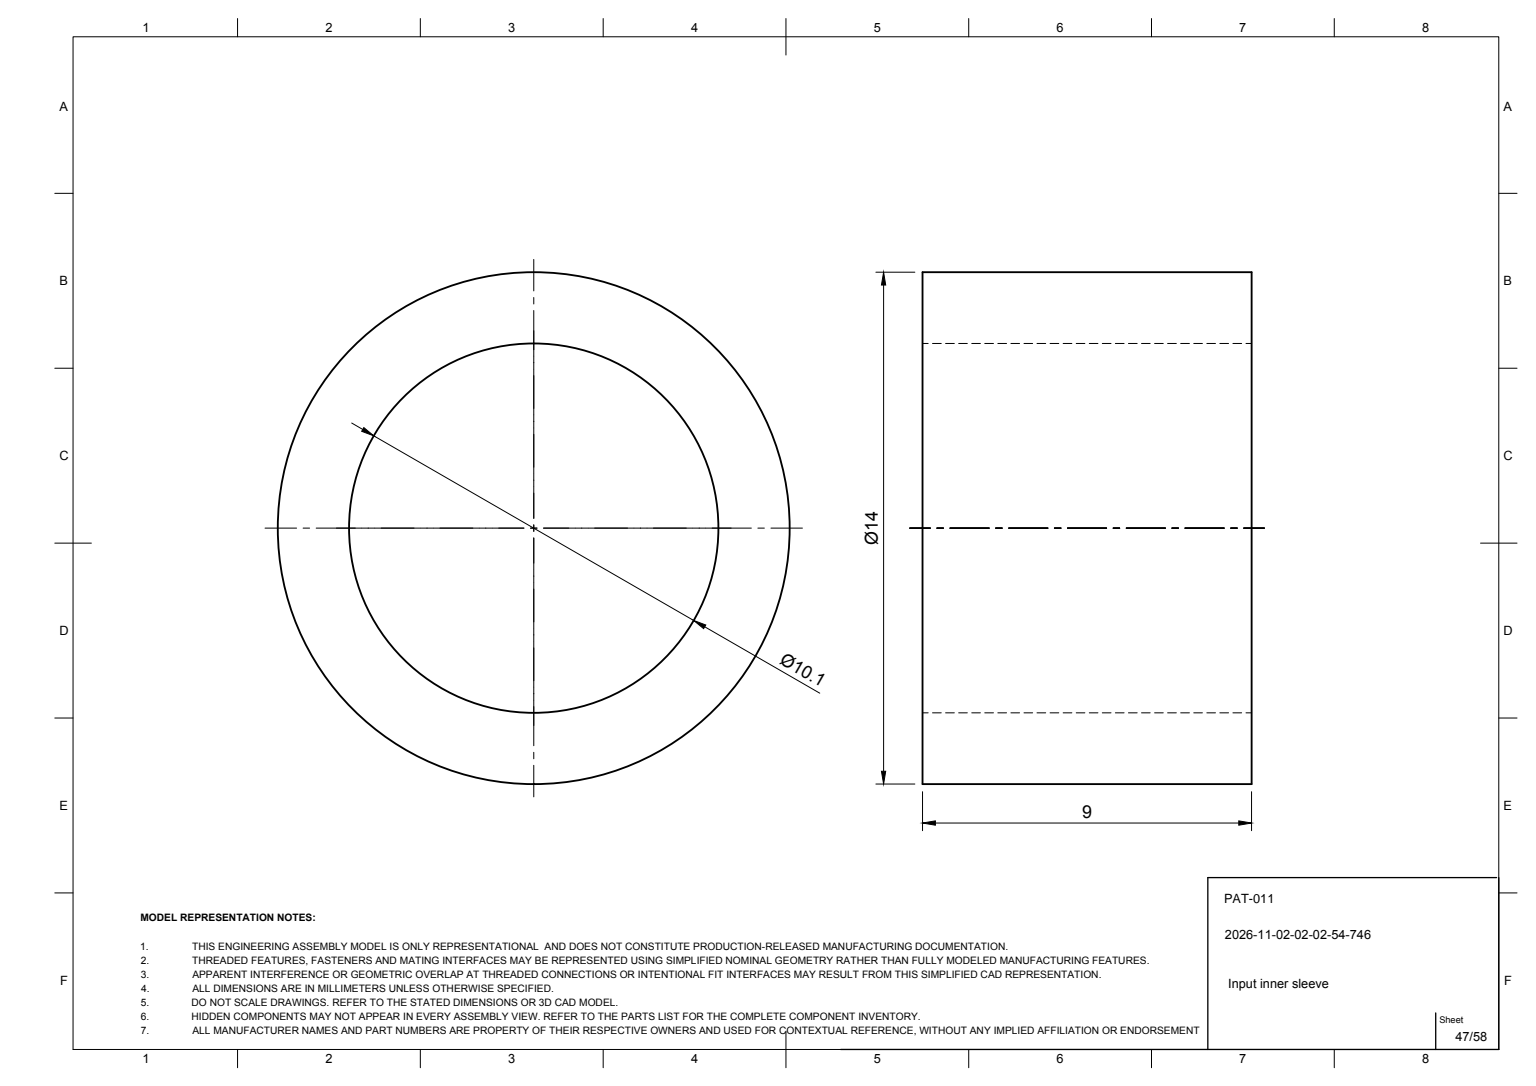
ISO-10303-21;
HEADER;
/* Generated by software containing ST-Developer
 * from STEP Tools, Inc. (www.steptools.com) 
 */

FILE_DESCRIPTION(
/* description */ ('Belt tension measurement rig'),
/* implementation_level */ '2;1');

FILE_NAME(
/* name */ 'Input inner sleeve.step',
/* time_stamp */ '2026-10-28T03:24:44-07:00',
/* author */ (''),
/* organization */ (''),
/* preprocessor_version */ 'ST-DEVELOPER v20.2',
/* originating_system */ 'Autodesk Translation Framework v15.17.0.0',
/* authorisation */ '');

FILE_SCHEMA (('AUTOMOTIVE_DESIGN { 1 0 10303 214 3 1 1 }'));
ENDSEC;

DATA;
#10=MECHANICAL_DESIGN_GEOMETRIC_PRESENTATION_REPRESENTATION('',(#746),#23587);
#621=SHAPE_REPRESENTATION_RELATIONSHIP('SRR','None',#23871,#676);
#676=ADVANCED_BREP_SHAPE_REPRESENTATION('',(#814),#23569);
#746=STYLED_ITEM('',(#24197),#814);
#814=MANIFOLD_SOLID_BREP('Body1',#12253);
#991=FACE_BOUND('',#2685,.T.);
#992=FACE_BOUND('',#2687,.T.);
#1286=PLANE('',#13848);
#1287=PLANE('',#13849);
#1816=FACE_OUTER_BOUND('',#2682,.T.);
#1817=FACE_OUTER_BOUND('',#2683,.T.);
#1818=FACE_OUTER_BOUND('',#2684,.T.);
#1819=FACE_OUTER_BOUND('',#2686,.T.);
#2682=EDGE_LOOP('',(#9968,#9969,#9970,#9971));
#2683=EDGE_LOOP('',(#9972,#9973,#9974,#9975));
#2684=EDGE_LOOP('',(#9976));
#2685=EDGE_LOOP('',(#9977));
#2686=EDGE_LOOP('',(#9978));
#2687=EDGE_LOOP('',(#9979));
#3501=LINE('',#21506,#4252);
#3502=LINE('',#21512,#4253);
#4252=VECTOR('',#16986,0.505);
#4253=VECTOR('',#16993,0.7);
#4912=CIRCLE('',#13843,0.505);
#4913=CIRCLE('',#13844,0.505);
#4914=CIRCLE('',#13846,0.7);
#4915=CIRCLE('',#13847,0.7);
#5927=VERTEX_POINT('',#21503);
#5928=VERTEX_POINT('',#21505);
#5929=VERTEX_POINT('',#21509);
#5930=VERTEX_POINT('',#21511);
#7343=EDGE_CURVE('',#5927,#5927,#4912,.T.);
#7344=EDGE_CURVE('',#5927,#5928,#3501,.T.);
#7345=EDGE_CURVE('',#5928,#5928,#4913,.T.);
#7346=EDGE_CURVE('',#5929,#5929,#4914,.T.);
#7347=EDGE_CURVE('',#5929,#5930,#3502,.T.);
#7348=EDGE_CURVE('',#5930,#5930,#4915,.T.);
#9968=ORIENTED_EDGE('',*,*,#7343,.F.);
#9969=ORIENTED_EDGE('',*,*,#7344,.T.);
#9970=ORIENTED_EDGE('',*,*,#7345,.T.);
#9971=ORIENTED_EDGE('',*,*,#7344,.F.);
#9972=ORIENTED_EDGE('',*,*,#7346,.F.);
#9973=ORIENTED_EDGE('',*,*,#7347,.T.);
#9974=ORIENTED_EDGE('',*,*,#7348,.T.);
#9975=ORIENTED_EDGE('',*,*,#7347,.F.);
#9976=ORIENTED_EDGE('',*,*,#7346,.T.);
#9977=ORIENTED_EDGE('',*,*,#7343,.T.);
#9978=ORIENTED_EDGE('',*,*,#7348,.F.);
#9979=ORIENTED_EDGE('',*,*,#7345,.F.);
#11325=CYLINDRICAL_SURFACE('',#13842,0.505);
#11326=CYLINDRICAL_SURFACE('',#13845,0.7);
#11957=ADVANCED_FACE('',(#1816),#11325,.F.);
#11958=ADVANCED_FACE('',(#1817),#11326,.T.);
#11959=ADVANCED_FACE('',(#1818,#991),#1286,.T.);
#11960=ADVANCED_FACE('',(#1819,#992),#1287,.F.);
#12253=CLOSED_SHELL('',(#11957,#11958,#11959,#11960));
#13841=AXIS2_PLACEMENT_3D('',#21501,#16980,#16981);
#13842=AXIS2_PLACEMENT_3D('',#21502,#16982,#16983);
#13843=AXIS2_PLACEMENT_3D('',#21504,#16984,#16985);
#13844=AXIS2_PLACEMENT_3D('',#21507,#16987,#16988);
#13845=AXIS2_PLACEMENT_3D('',#21508,#16989,#16990);
#13846=AXIS2_PLACEMENT_3D('',#21510,#16991,#16992);
#13847=AXIS2_PLACEMENT_3D('',#21513,#16994,#16995);
#13848=AXIS2_PLACEMENT_3D('',#21514,#16996,#16997);
#13849=AXIS2_PLACEMENT_3D('',#21515,#16998,#16999);
#16980=DIRECTION('axis',(0.,0.,1.));
#16981=DIRECTION('refdir',(1.,0.,0.));
#16982=DIRECTION('center_axis',(0.,1.,0.));
#16983=DIRECTION('ref_axis',(1.,0.,0.));
#16984=DIRECTION('center_axis',(0.,-1.,0.));
#16985=DIRECTION('ref_axis',(1.,0.,0.));
#16986=DIRECTION('',(0.,-1.,0.));
#16987=DIRECTION('center_axis',(0.,-1.,0.));
#16988=DIRECTION('ref_axis',(1.,0.,0.));
#16989=DIRECTION('center_axis',(0.,1.,0.));
#16990=DIRECTION('ref_axis',(1.,0.,0.));
#16991=DIRECTION('center_axis',(0.,1.,0.));
#16992=DIRECTION('ref_axis',(1.,0.,0.));
#16993=DIRECTION('',(0.,-1.,0.));
#16994=DIRECTION('center_axis',(0.,1.,0.));
#16995=DIRECTION('ref_axis',(1.,0.,0.));
#16996=DIRECTION('center_axis',(0.,1.,0.));
#16997=DIRECTION('ref_axis',(1.,0.,0.));
#16998=DIRECTION('center_axis',(0.,1.,0.));
#16999=DIRECTION('ref_axis',(1.,0.,0.));
#21501=CARTESIAN_POINT('',(0.,0.,0.));
#21502=CARTESIAN_POINT('Origin',(0.,-0.45,7.));
#21503=CARTESIAN_POINT('',(-0.505,0.45,7.));
#21504=CARTESIAN_POINT('Origin',(0.,0.45,7.));
#21505=CARTESIAN_POINT('',(-0.505,-0.45,7.));
#21506=CARTESIAN_POINT('',(-0.505,-0.45,7.));
#21507=CARTESIAN_POINT('Origin',(0.,-0.45,7.));
#21508=CARTESIAN_POINT('Origin',(0.,-0.45,7.));
#21509=CARTESIAN_POINT('',(-0.7,0.45,7.));
#21510=CARTESIAN_POINT('Origin',(0.,0.45,7.));
#21511=CARTESIAN_POINT('',(-0.7,-0.45,7.));
#21512=CARTESIAN_POINT('',(-0.7,-0.45,7.));
#21513=CARTESIAN_POINT('Origin',(0.,-0.45,7.));
#21514=CARTESIAN_POINT('Origin',(0.,0.45,7.));
#21515=CARTESIAN_POINT('Origin',(0.,-0.45,7.));
#23504=UNCERTAINTY_MEASURE_WITH_UNIT(LENGTH_MEASURE(0.001),#23588,
'DISTANCE_ACCURACY_VALUE',
'Maximum model space distance between geometric entities at asserted c
onnectivities');
#23522=UNCERTAINTY_MEASURE_WITH_UNIT(LENGTH_MEASURE(0.001),#23588,
'DISTANCE_ACCURACY_VALUE',
'Maximum model space distance between geometric entities at asserted c
onnectivities');
#23569=(
GEOMETRIC_REPRESENTATION_CONTEXT(3)
GLOBAL_UNCERTAINTY_ASSIGNED_CONTEXT((#23504))
GLOBAL_UNIT_ASSIGNED_CONTEXT((#23588,#23590,#23591))
REPRESENTATION_CONTEXT('','3D')
);
#23587=(
GEOMETRIC_REPRESENTATION_CONTEXT(3)
GLOBAL_UNCERTAINTY_ASSIGNED_CONTEXT((#23522))
GLOBAL_UNIT_ASSIGNED_CONTEXT((#23588,#23590,#23591))
REPRESENTATION_CONTEXT('','3D')
);
#23588=(
LENGTH_UNIT()
NAMED_UNIT(*)
SI_UNIT(.CENTI.,.METRE.)
);
#23590=(
NAMED_UNIT(*)
PLANE_ANGLE_UNIT()
SI_UNIT($,.RADIAN.)
);
#23591=(
NAMED_UNIT(*)
SI_UNIT($,.STERADIAN.)
SOLID_ANGLE_UNIT()
);
#23638=SHAPE_DEFINITION_REPRESENTATION(#23715,#23871);
#23715=PRODUCT_DEFINITION_SHAPE('',$,#23936);
#23871=SHAPE_REPRESENTATION('',(#13841),#23569);
#23889=PRODUCT_DEFINITION_CONTEXT('part definition',#24083,'design');
#23936=PRODUCT_DEFINITION('Input inner sleeve','Input inner sleeve',#24000,
#23889);
#24000=PRODUCT_DEFINITION_FORMATION('',$,#24131);
#24083=APPLICATION_CONTEXT(
'Core Data for Automotive Mechanical Design Process');
#24084=PRODUCT_CONTEXT('part definition',#24083,'mechanical');
#24131=PRODUCT('Input inner sleeve','Input inner sleeve',
'Input inner sleeve',(#24084));
#24191=COLOUR_RGB('Light Blue',0.38,0.62,0.78);
#24192=FILL_AREA_STYLE_COLOUR('',#24191);
#24193=FILL_AREA_STYLE('',(#24192));
#24194=SURFACE_STYLE_FILL_AREA(#24193);
#24195=SURFACE_SIDE_STYLE('',(#24194));
#24196=SURFACE_STYLE_USAGE(.BOTH.,#24195);
#24197=PRESENTATION_STYLE_ASSIGNMENT((#24196));
ENDSEC;
END-ISO-10303-21;
